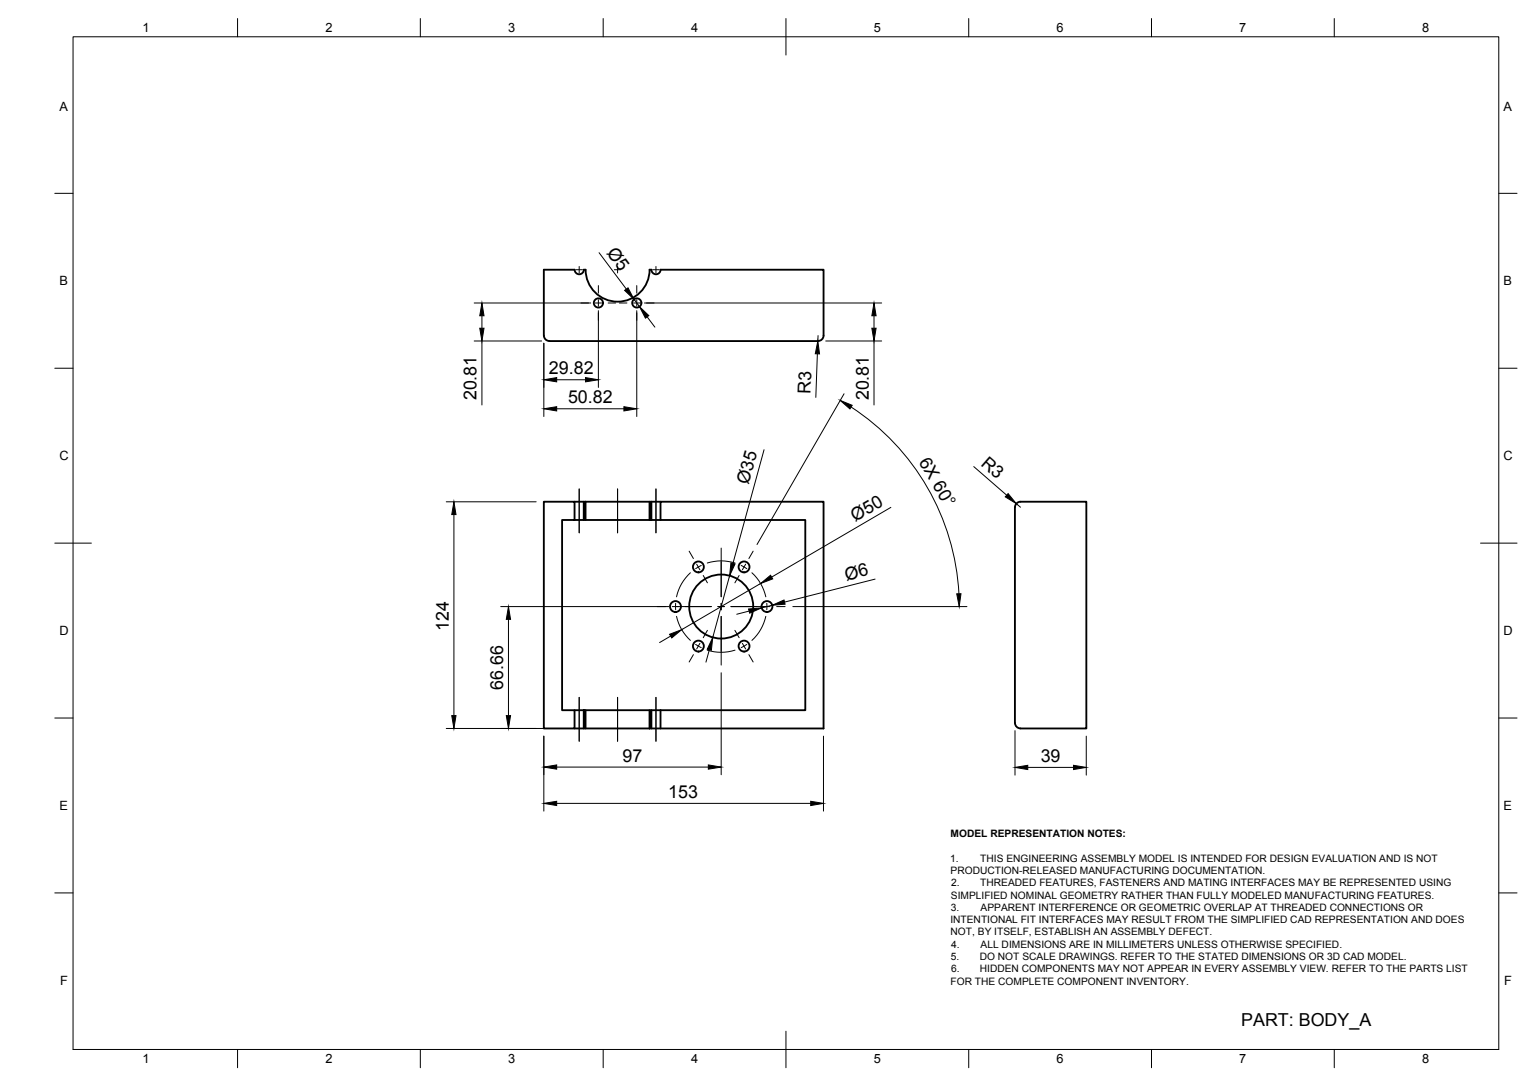
ISO-10303-21;
HEADER;
/* Generated by software containing ST-Developer
 * from STEP Tools, Inc. (www.steptools.com) 
 */

FILE_DESCRIPTION(
/* description */ ('STEP AP214'),
/* implementation_level */ '2;1');

FILE_NAME(
/* name */ 'Body_A.step',
/* time_stamp */ '2026-10-05T13:15:56-07:00',
/* author */ (''),
/* organization */ (''),
/* preprocessor_version */ 'ST-DEVELOPER v20.2',
/* originating_system */ 'Autodesk Translation Framework v15.15.0.0',
/* authorisation */ '');

FILE_SCHEMA (('AUTOMOTIVE_DESIGN { 1 0 10303 214 3 1 1 }'));
ENDSEC;

DATA;
#10=MECHANICAL_DESIGN_GEOMETRIC_PRESENTATION_REPRESENTATION('',(#1345),#37881);
#1321=SHAPE_REPRESENTATION_RELATIONSHIP('SRR','None',#37954,#1333);
#1333=ADVANCED_BREP_SHAPE_REPRESENTATION('',(#1357),#37869);
#1345=STYLED_ITEM('',(#38023),#1357);
#1357=MANIFOLD_SOLID_BREP('Body1',#10819);
#1369=ELLIPSE('',#11034,4.24264068711896,2.99999999999969);
#1370=ELLIPSE('',#11035,4.24264068711823,2.99999999999929);
#1371=ELLIPSE('',#11037,4.24264068711881,2.99999999999963);
#1372=ELLIPSE('',#11039,4.24264068711841,2.99999999999935);
#1377=FACE_BOUND('',#2191,.T.);
#1378=FACE_BOUND('',#2192,.T.);
#1379=FACE_BOUND('',#2195,.T.);
#1380=FACE_BOUND('',#2196,.T.);
#1381=FACE_BOUND('',#2200,.T.);
#1382=FACE_BOUND('',#2201,.T.);
#1383=FACE_BOUND('',#2204,.T.);
#1384=FACE_BOUND('',#2205,.T.);
#1385=FACE_BOUND('',#2208,.T.);
#1386=FACE_BOUND('',#2209,.T.);
#1387=FACE_BOUND('',#2210,.T.);
#1388=FACE_BOUND('',#2211,.T.);
#1389=FACE_BOUND('',#2212,.T.);
#1390=FACE_BOUND('',#2213,.T.);
#1391=FACE_BOUND('',#2214,.T.);
#1392=FACE_BOUND('',#2216,.T.);
#1393=FACE_BOUND('',#2217,.T.);
#1394=FACE_BOUND('',#2218,.T.);
#1395=FACE_BOUND('',#2219,.T.);
#1396=FACE_BOUND('',#2220,.T.);
#1397=FACE_BOUND('',#2221,.T.);
#1398=FACE_BOUND('',#2222,.T.);
#1465=PLANE('',#10999);
#1466=PLANE('',#11000);
#1467=PLANE('',#11001);
#1468=PLANE('',#11002);
#1469=PLANE('',#11003);
#1470=PLANE('',#11004);
#1471=PLANE('',#11008);
#1472=PLANE('',#11009);
#1473=PLANE('',#11013);
#1474=PLANE('',#11014);
#1475=PLANE('',#11015);
#1476=PLANE('',#11019);
#1477=PLANE('',#11020);
#1478=PLANE('',#11024);
#1479=PLANE('',#11025);
#1480=PLANE('',#11026);
#1565=FACE_OUTER_BOUND('',#2174,.T.);
#1566=FACE_OUTER_BOUND('',#2175,.T.);
#1567=FACE_OUTER_BOUND('',#2176,.T.);
#1568=FACE_OUTER_BOUND('',#2177,.T.);
#1569=FACE_OUTER_BOUND('',#2178,.T.);
#1570=FACE_OUTER_BOUND('',#2179,.T.);
#1571=FACE_OUTER_BOUND('',#2180,.T.);
#1572=FACE_OUTER_BOUND('',#2181,.T.);
#1573=FACE_OUTER_BOUND('',#2182,.T.);
#1574=FACE_OUTER_BOUND('',#2183,.T.);
#1575=FACE_OUTER_BOUND('',#2184,.T.);
#1576=FACE_OUTER_BOUND('',#2185,.T.);
#1577=FACE_OUTER_BOUND('',#2186,.T.);
#1578=FACE_OUTER_BOUND('',#2187,.T.);
#1579=FACE_OUTER_BOUND('',#2188,.T.);
#1580=FACE_OUTER_BOUND('',#2189,.T.);
#1581=FACE_OUTER_BOUND('',#2190,.T.);
#1582=FACE_OUTER_BOUND('',#2193,.T.);
#1583=FACE_OUTER_BOUND('',#2194,.T.);
#1584=FACE_OUTER_BOUND('',#2197,.T.);
#1585=FACE_OUTER_BOUND('',#2198,.T.);
#1586=FACE_OUTER_BOUND('',#2199,.T.);
#1587=FACE_OUTER_BOUND('',#2202,.T.);
#1588=FACE_OUTER_BOUND('',#2203,.T.);
#1589=FACE_OUTER_BOUND('',#2206,.T.);
#1590=FACE_OUTER_BOUND('',#2207,.T.);
#1591=FACE_OUTER_BOUND('',#2215,.T.);
#1592=FACE_OUTER_BOUND('',#2223,.T.);
#1593=FACE_OUTER_BOUND('',#2224,.T.);
#1594=FACE_OUTER_BOUND('',#2225,.T.);
#1595=FACE_OUTER_BOUND('',#2226,.T.);
#1596=FACE_OUTER_BOUND('',#2227,.T.);
#1597=FACE_OUTER_BOUND('',#2228,.T.);
#1598=FACE_OUTER_BOUND('',#2229,.T.);
#1599=FACE_OUTER_BOUND('',#2230,.T.);
#1600=FACE_OUTER_BOUND('',#2231,.T.);
#1601=FACE_OUTER_BOUND('',#2232,.T.);
#2174=EDGE_LOOP('',(#6725,#6726,#6727,#6728));
#2175=EDGE_LOOP('',(#6729,#6730,#6731,#6732));
#2176=EDGE_LOOP('',(#6733,#6734,#6735,#6736));
#2177=EDGE_LOOP('',(#6737,#6738,#6739,#6740));
#2178=EDGE_LOOP('',(#6741,#6742,#6743,#6744));
#2179=EDGE_LOOP('',(#6745,#6746,#6747,#6748));
#2180=EDGE_LOOP('',(#6749,#6750,#6751,#6752));
#2181=EDGE_LOOP('',(#6753,#6754,#6755,#6756));
#2182=EDGE_LOOP('',(#6757,#6758,#6759,#6760));
#2183=EDGE_LOOP('',(#6761,#6762,#6763,#6764));
#2184=EDGE_LOOP('',(#6765,#6766,#6767,#6768));
#2185=EDGE_LOOP('',(#6769,#6770,#6771,#6772,#6773,#6774,#6775,#6776));
#2186=EDGE_LOOP('',(#6777,#6778,#6779,#6780));
#2187=EDGE_LOOP('',(#6781,#6782,#6783,#6784));
#2188=EDGE_LOOP('',(#6785,#6786,#6787,#6788));
#2189=EDGE_LOOP('',(#6789,#6790,#6791,#6792));
#2190=EDGE_LOOP('',(#6793,#6794,#6795,#6796,#6797,#6798,#6799,#6800,#6801,
#6802));
#2191=EDGE_LOOP('',(#6803));
#2192=EDGE_LOOP('',(#6804));
#2193=EDGE_LOOP('',(#6805,#6806,#6807,#6808,#6809,#6810,#6811,#6812));
#2194=EDGE_LOOP('',(#6813,#6814,#6815,#6816,#6817,#6818,#6819,#6820,#6821,
#6822));
#2195=EDGE_LOOP('',(#6823));
#2196=EDGE_LOOP('',(#6824));
#2197=EDGE_LOOP('',(#6825,#6826,#6827,#6828));
#2198=EDGE_LOOP('',(#6829,#6830,#6831,#6832));
#2199=EDGE_LOOP('',(#6833,#6834,#6835,#6836,#6837,#6838,#6839,#6840,#6841,
#6842));
#2200=EDGE_LOOP('',(#6843));
#2201=EDGE_LOOP('',(#6844));
#2202=EDGE_LOOP('',(#6845,#6846,#6847,#6848));
#2203=EDGE_LOOP('',(#6849,#6850,#6851,#6852,#6853,#6854,#6855,#6856,#6857,
#6858));
#2204=EDGE_LOOP('',(#6859));
#2205=EDGE_LOOP('',(#6860));
#2206=EDGE_LOOP('',(#6861,#6862,#6863,#6864));
#2207=EDGE_LOOP('',(#6865,#6866,#6867,#6868));
#2208=EDGE_LOOP('',(#6869));
#2209=EDGE_LOOP('',(#6870));
#2210=EDGE_LOOP('',(#6871));
#2211=EDGE_LOOP('',(#6872));
#2212=EDGE_LOOP('',(#6873));
#2213=EDGE_LOOP('',(#6874));
#2214=EDGE_LOOP('',(#6875));
#2215=EDGE_LOOP('',(#6876,#6877,#6878,#6879));
#2216=EDGE_LOOP('',(#6880));
#2217=EDGE_LOOP('',(#6881));
#2218=EDGE_LOOP('',(#6882));
#2219=EDGE_LOOP('',(#6883));
#2220=EDGE_LOOP('',(#6884));
#2221=EDGE_LOOP('',(#6885));
#2222=EDGE_LOOP('',(#6886));
#2223=EDGE_LOOP('',(#6887,#6888,#6889,#6890));
#2224=EDGE_LOOP('',(#6891,#6892,#6893,#6894));
#2225=EDGE_LOOP('',(#6895,#6896,#6897,#6898));
#2226=EDGE_LOOP('',(#6899,#6900,#6901,#6902));
#2227=EDGE_LOOP('',(#6903,#6904,#6905,#6906));
#2228=EDGE_LOOP('',(#6907,#6908,#6909,#6910));
#2229=EDGE_LOOP('',(#6911,#6912,#6913,#6914));
#2230=EDGE_LOOP('',(#6915,#6916,#6917,#6918));
#2231=EDGE_LOOP('',(#6919,#6920,#6921,#6922));
#2232=EDGE_LOOP('',(#6923,#6924,#6925,#6926));
#2871=LINE('',#14049,#3172);
#2872=LINE('',#14055,#3173);
#2873=LINE('',#14061,#3174);
#2874=LINE('',#14067,#3175);
#2875=LINE('',#14073,#3176);
#2876=LINE('',#14079,#3177);
#2877=LINE('',#14085,#3178);
#2878=LINE('',#14091,#3179);
#2879=LINE('',#14097,#3180);
#2880=LINE('',#14103,#3181);
#2881=LINE('',#14109,#3182);
#2882=LINE('',#14114,#3183);
#2883=LINE('',#14116,#3184);
#2884=LINE('',#14118,#3185);
#2885=LINE('',#14120,#3186);
#2886=LINE('',#14122,#3187);
#2887=LINE('',#14124,#3188);
#2888=LINE('',#14126,#3189);
#2889=LINE('',#14127,#3190);
#2890=LINE('',#14131,#3191);
#2891=LINE('',#14133,#3192);
#2892=LINE('',#14135,#3193);
#2893=LINE('',#14136,#3194);
#2894=LINE('',#14140,#3195);
#2895=LINE('',#14142,#3196);
#2896=LINE('',#14144,#3197);
#2897=LINE('',#14145,#3198);
#2898=LINE('',#14149,#3199);
#2899=LINE('',#14151,#3200);
#2900=LINE('',#14153,#3201);
#2901=LINE('',#14154,#3202);
#2902=LINE('',#14158,#3203);
#2903=LINE('',#14160,#3204);
#2904=LINE('',#14162,#3205);
#2905=LINE('',#14163,#3206);
#2906=LINE('',#14166,#3207);
#2907=LINE('',#14168,#3208);
#2908=LINE('',#14170,#3209);
#2909=LINE('',#14172,#3210);
#2910=LINE('',#14178,#3211);
#2911=LINE('',#14180,#3212);
#2912=LINE('',#14182,#3213);
#2913=LINE('',#14184,#3214);
#2914=LINE('',#14186,#3215);
#2915=LINE('',#14188,#3216);
#2916=LINE('',#14189,#3217);
#2917=LINE('',#14192,#3218);
#2918=LINE('',#14194,#3219);
#2919=LINE('',#14195,#3220);
#2920=LINE('',#14200,#3221);
#2921=LINE('',#14202,#3222);
#2922=LINE('',#14208,#3223);
#2923=LINE('',#14210,#3224);
#2924=LINE('',#14211,#3225);
#2925=LINE('',#14214,#3226);
#2926=LINE('',#14215,#3227);
#2927=LINE('',#14219,#3228);
#2928=LINE('',#14220,#3229);
#2929=LINE('',#14224,#3230);
#2930=LINE('',#14229,#3231);
#2931=LINE('',#14231,#3232);
#2932=LINE('',#14233,#3233);
#2933=LINE('',#14234,#3234);
#3172=VECTOR('',#11898,2.5);
#3173=VECTOR('',#11905,2.5);
#3174=VECTOR('',#11912,2.5);
#3175=VECTOR('',#11919,2.5);
#3176=VECTOR('',#11926,3.);
#3177=VECTOR('',#11933,2.99999999999999);
#3178=VECTOR('',#11940,3.);
#3179=VECTOR('',#11947,3.);
#3180=VECTOR('',#11954,3.);
#3181=VECTOR('',#11961,3.);
#3182=VECTOR('',#11968,17.5);
#3183=VECTOR('',#11973,1000.);
#3184=VECTOR('',#11974,1000.);
#3185=VECTOR('',#11975,1000.);
#3186=VECTOR('',#11976,1000.);
#3187=VECTOR('',#11977,1000.);
#3188=VECTOR('',#11978,1000.);
#3189=VECTOR('',#11979,1000.);
#3190=VECTOR('',#11980,1000.);
#3191=VECTOR('',#11983,1000.);
#3192=VECTOR('',#11984,1000.);
#3193=VECTOR('',#11985,1000.);
#3194=VECTOR('',#11986,1000.);
#3195=VECTOR('',#11989,1000.);
#3196=VECTOR('',#11990,1000.);
#3197=VECTOR('',#11991,1000.);
#3198=VECTOR('',#11992,1000.);
#3199=VECTOR('',#11995,1000.);
#3200=VECTOR('',#11996,1000.);
#3201=VECTOR('',#11997,1000.);
#3202=VECTOR('',#11998,1000.);
#3203=VECTOR('',#12001,1000.);
#3204=VECTOR('',#12002,1000.);
#3205=VECTOR('',#12003,1000.);
#3206=VECTOR('',#12004,1000.);
#3207=VECTOR('',#12007,1000.);
#3208=VECTOR('',#12008,1000.);
#3209=VECTOR('',#12009,1000.);
#3210=VECTOR('',#12010,1000.);
#3211=VECTOR('',#12019,1000.);
#3212=VECTOR('',#12020,1000.);
#3213=VECTOR('',#12021,1000.);
#3214=VECTOR('',#12022,1000.);
#3215=VECTOR('',#12023,1000.);
#3216=VECTOR('',#12024,1000.);
#3217=VECTOR('',#12025,1000.);
#3218=VECTOR('',#12028,1000.);
#3219=VECTOR('',#12029,1000.);
#3220=VECTOR('',#12030,1000.);
#3221=VECTOR('',#12039,1000.);
#3222=VECTOR('',#12042,1000.);
#3223=VECTOR('',#12051,1000.);
#3224=VECTOR('',#12052,1000.);
#3225=VECTOR('',#12053,1000.);
#3226=VECTOR('',#12056,1000.);
#3227=VECTOR('',#12057,1000.);
#3228=VECTOR('',#12062,1000.);
#3229=VECTOR('',#12063,1000.);
#3230=VECTOR('',#12070,1000.);
#3231=VECTOR('',#12075,1000.);
#3232=VECTOR('',#12076,1000.);
#3233=VECTOR('',#12077,1000.);
#3234=VECTOR('',#12078,1000.);
#3473=CIRCLE('',#10967,2.5);
#3474=CIRCLE('',#10968,2.5);
#3475=CIRCLE('',#10970,2.5);
#3476=CIRCLE('',#10971,2.5);
#3477=CIRCLE('',#10973,2.5);
#3478=CIRCLE('',#10974,2.5);
#3479=CIRCLE('',#10976,2.5);
#3480=CIRCLE('',#10977,2.5);
#3481=CIRCLE('',#10979,3.);
#3482=CIRCLE('',#10980,3.);
#3483=CIRCLE('',#10982,2.99999999999999);
#3484=CIRCLE('',#10983,2.99999999999999);
#3485=CIRCLE('',#10985,3.);
#3486=CIRCLE('',#10986,3.);
#3487=CIRCLE('',#10988,3.);
#3488=CIRCLE('',#10989,3.);
#3489=CIRCLE('',#10991,3.);
#3490=CIRCLE('',#10992,3.);
#3491=CIRCLE('',#10994,3.);
#3492=CIRCLE('',#10995,3.);
#3493=CIRCLE('',#10997,17.5);
#3494=CIRCLE('',#10998,17.5);
#3495=CIRCLE('',#11005,2.50000000000001);
#3496=CIRCLE('',#11006,17.5);
#3497=CIRCLE('',#11007,2.5);
#3498=CIRCLE('',#11010,2.5);
#3499=CIRCLE('',#11011,17.5);
#3500=CIRCLE('',#11012,2.50000000000001);
#3501=CIRCLE('',#11016,2.5);
#3502=CIRCLE('',#11017,17.5);
#3503=CIRCLE('',#11018,2.50000000000001);
#3504=CIRCLE('',#11021,2.5);
#3505=CIRCLE('',#11022,2.50000000000001);
#3506=CIRCLE('',#11023,17.5);
#3998=VERTEX_POINT('',#14046);
#3999=VERTEX_POINT('',#14048);
#4000=VERTEX_POINT('',#14052);
#4001=VERTEX_POINT('',#14054);
#4002=VERTEX_POINT('',#14058);
#4003=VERTEX_POINT('',#14060);
#4004=VERTEX_POINT('',#14064);
#4005=VERTEX_POINT('',#14066);
#4006=VERTEX_POINT('',#14070);
#4007=VERTEX_POINT('',#14072);
#4008=VERTEX_POINT('',#14076);
#4009=VERTEX_POINT('',#14078);
#4010=VERTEX_POINT('',#14082);
#4011=VERTEX_POINT('',#14084);
#4012=VERTEX_POINT('',#14088);
#4013=VERTEX_POINT('',#14090);
#4014=VERTEX_POINT('',#14094);
#4015=VERTEX_POINT('',#14096);
#4016=VERTEX_POINT('',#14100);
#4017=VERTEX_POINT('',#14102);
#4018=VERTEX_POINT('',#14106);
#4019=VERTEX_POINT('',#14108);
#4020=VERTEX_POINT('',#14112);
#4021=VERTEX_POINT('',#14113);
#4022=VERTEX_POINT('',#14115);
#4023=VERTEX_POINT('',#14117);
#4024=VERTEX_POINT('',#14119);
#4025=VERTEX_POINT('',#14121);
#4026=VERTEX_POINT('',#14123);
#4027=VERTEX_POINT('',#14125);
#4028=VERTEX_POINT('',#14129);
#4029=VERTEX_POINT('',#14130);
#4030=VERTEX_POINT('',#14132);
#4031=VERTEX_POINT('',#14134);
#4032=VERTEX_POINT('',#14138);
#4033=VERTEX_POINT('',#14139);
#4034=VERTEX_POINT('',#14141);
#4035=VERTEX_POINT('',#14143);
#4036=VERTEX_POINT('',#14147);
#4037=VERTEX_POINT('',#14148);
#4038=VERTEX_POINT('',#14150);
#4039=VERTEX_POINT('',#14152);
#4040=VERTEX_POINT('',#14156);
#4041=VERTEX_POINT('',#14157);
#4042=VERTEX_POINT('',#14159);
#4043=VERTEX_POINT('',#14161);
#4044=VERTEX_POINT('',#14165);
#4045=VERTEX_POINT('',#14167);
#4046=VERTEX_POINT('',#14169);
#4047=VERTEX_POINT('',#14171);
#4048=VERTEX_POINT('',#14177);
#4049=VERTEX_POINT('',#14179);
#4050=VERTEX_POINT('',#14181);
#4051=VERTEX_POINT('',#14183);
#4052=VERTEX_POINT('',#14185);
#4053=VERTEX_POINT('',#14187);
#4054=VERTEX_POINT('',#14191);
#4055=VERTEX_POINT('',#14193);
#4056=VERTEX_POINT('',#14207);
#4057=VERTEX_POINT('',#14209);
#4058=VERTEX_POINT('',#14213);
#4059=VERTEX_POINT('',#14218);
#4060=VERTEX_POINT('',#14227);
#4061=VERTEX_POINT('',#14228);
#4062=VERTEX_POINT('',#14230);
#4063=VERTEX_POINT('',#14232);
#5073=EDGE_CURVE('',#3998,#3998,#3473,.T.);
#5074=EDGE_CURVE('',#3998,#3999,#2871,.T.);
#5075=EDGE_CURVE('',#3999,#3999,#3474,.T.);
#5076=EDGE_CURVE('',#4000,#4000,#3475,.T.);
#5077=EDGE_CURVE('',#4000,#4001,#2872,.T.);
#5078=EDGE_CURVE('',#4001,#4001,#3476,.T.);
#5079=EDGE_CURVE('',#4002,#4002,#3477,.T.);
#5080=EDGE_CURVE('',#4002,#4003,#2873,.T.);
#5081=EDGE_CURVE('',#4003,#4003,#3478,.T.);
#5082=EDGE_CURVE('',#4004,#4004,#3479,.T.);
#5083=EDGE_CURVE('',#4004,#4005,#2874,.T.);
#5084=EDGE_CURVE('',#4005,#4005,#3480,.T.);
#5085=EDGE_CURVE('',#4006,#4006,#3481,.T.);
#5086=EDGE_CURVE('',#4006,#4007,#2875,.T.);
#5087=EDGE_CURVE('',#4007,#4007,#3482,.T.);
#5088=EDGE_CURVE('',#4008,#4008,#3483,.T.);
#5089=EDGE_CURVE('',#4008,#4009,#2876,.T.);
#5090=EDGE_CURVE('',#4009,#4009,#3484,.T.);
#5091=EDGE_CURVE('',#4010,#4010,#3485,.T.);
#5092=EDGE_CURVE('',#4010,#4011,#2877,.T.);
#5093=EDGE_CURVE('',#4011,#4011,#3486,.T.);
#5094=EDGE_CURVE('',#4012,#4012,#3487,.T.);
#5095=EDGE_CURVE('',#4012,#4013,#2878,.T.);
#5096=EDGE_CURVE('',#4013,#4013,#3488,.T.);
#5097=EDGE_CURVE('',#4014,#4014,#3489,.T.);
#5098=EDGE_CURVE('',#4014,#4015,#2879,.T.);
#5099=EDGE_CURVE('',#4015,#4015,#3490,.T.);
#5100=EDGE_CURVE('',#4016,#4016,#3491,.T.);
#5101=EDGE_CURVE('',#4016,#4017,#2880,.T.);
#5102=EDGE_CURVE('',#4017,#4017,#3492,.T.);
#5103=EDGE_CURVE('',#4018,#4018,#3493,.T.);
#5104=EDGE_CURVE('',#4018,#4019,#2881,.T.);
#5105=EDGE_CURVE('',#4019,#4019,#3494,.T.);
#5106=EDGE_CURVE('',#4020,#4021,#2882,.T.);
#5107=EDGE_CURVE('',#4022,#4020,#2883,.T.);
#5108=EDGE_CURVE('',#4023,#4022,#2884,.T.);
#5109=EDGE_CURVE('',#4024,#4023,#2885,.T.);
#5110=EDGE_CURVE('',#4025,#4024,#2886,.T.);
#5111=EDGE_CURVE('',#4025,#4026,#2887,.T.);
#5112=EDGE_CURVE('',#4026,#4027,#2888,.T.);
#5113=EDGE_CURVE('',#4027,#4021,#2889,.T.);
#5114=EDGE_CURVE('',#4028,#4029,#2890,.T.);
#5115=EDGE_CURVE('',#4030,#4028,#2891,.T.);
#5116=EDGE_CURVE('',#4031,#4030,#2892,.T.);
#5117=EDGE_CURVE('',#4031,#4029,#2893,.T.);
#5118=EDGE_CURVE('',#4032,#4033,#2894,.T.);
#5119=EDGE_CURVE('',#4032,#4034,#2895,.T.);
#5120=EDGE_CURVE('',#4035,#4034,#2896,.T.);
#5121=EDGE_CURVE('',#4033,#4035,#2897,.T.);
#5122=EDGE_CURVE('',#4036,#4037,#2898,.T.);
#5123=EDGE_CURVE('',#4038,#4036,#2899,.T.);
#5124=EDGE_CURVE('',#4039,#4038,#2900,.T.);
#5125=EDGE_CURVE('',#4039,#4037,#2901,.T.);
#5126=EDGE_CURVE('',#4040,#4041,#2902,.T.);
#5127=EDGE_CURVE('',#4040,#4042,#2903,.T.);
#5128=EDGE_CURVE('',#4043,#4042,#2904,.T.);
#5129=EDGE_CURVE('',#4041,#4043,#2905,.T.);
#5130=EDGE_CURVE('',#4044,#4023,#2906,.T.);
#5131=EDGE_CURVE('',#4044,#4045,#2907,.T.);
#5132=EDGE_CURVE('',#4045,#4046,#2908,.T.);
#5133=EDGE_CURVE('',#4046,#4047,#2909,.T.);
#5134=EDGE_CURVE('',#4033,#4047,#3495,.T.);
#5135=EDGE_CURVE('',#4030,#4035,#3496,.T.);
#5136=EDGE_CURVE('',#4024,#4028,#3497,.T.);
#5137=EDGE_CURVE('',#4047,#4048,#2910,.T.);
#5138=EDGE_CURVE('',#4049,#4046,#2911,.T.);
#5139=EDGE_CURVE('',#4050,#4049,#2912,.T.);
#5140=EDGE_CURVE('',#4051,#4050,#2913,.T.);
#5141=EDGE_CURVE('',#4051,#4052,#2914,.T.);
#5142=EDGE_CURVE('',#4052,#4053,#2915,.T.);
#5143=EDGE_CURVE('',#4053,#4048,#2916,.T.);
#5144=EDGE_CURVE('',#4054,#4049,#2917,.T.);
#5145=EDGE_CURVE('',#4054,#4055,#2918,.T.);
#5146=EDGE_CURVE('',#4055,#4022,#2919,.T.);
#5147=EDGE_CURVE('',#4020,#4041,#3498,.T.);
#5148=EDGE_CURVE('',#4043,#4038,#3499,.T.);
#5149=EDGE_CURVE('',#4036,#4050,#3500,.T.);
#5150=EDGE_CURVE('',#4045,#4054,#2920,.T.);
#5151=EDGE_CURVE('',#4055,#4044,#2921,.T.);
#5152=EDGE_CURVE('',#4029,#4025,#3501,.T.);
#5153=EDGE_CURVE('',#4034,#4031,#3502,.T.);
#5154=EDGE_CURVE('',#4048,#4032,#3503,.T.);
#5155=EDGE_CURVE('',#4056,#4053,#2922,.T.);
#5156=EDGE_CURVE('',#4056,#4057,#2923,.T.);
#5157=EDGE_CURVE('',#4057,#4026,#2924,.T.);
#5158=EDGE_CURVE('',#4057,#4058,#2925,.T.);
#5159=EDGE_CURVE('',#4058,#4027,#2926,.T.);
#5160=EDGE_CURVE('',#4021,#4040,#3504,.T.);
#5161=EDGE_CURVE('',#4058,#4059,#2927,.T.);
#5162=EDGE_CURVE('',#4059,#4052,#2928,.T.);
#5163=EDGE_CURVE('',#4037,#4051,#3505,.T.);
#5164=EDGE_CURVE('',#4042,#4039,#3506,.T.);
#5165=EDGE_CURVE('',#4059,#4056,#2929,.T.);
#5166=EDGE_CURVE('',#4060,#4061,#2930,.T.);
#5167=EDGE_CURVE('',#4061,#4062,#2931,.T.);
#5168=EDGE_CURVE('',#4062,#4063,#2932,.T.);
#5169=EDGE_CURVE('',#4063,#4060,#2933,.T.);
#5170=EDGE_CURVE('',#4045,#4063,#1369,.T.);
#5171=EDGE_CURVE('',#4060,#4044,#1370,.T.);
#5172=EDGE_CURVE('',#4061,#4055,#1371,.T.);
#5173=EDGE_CURVE('',#4054,#4062,#1372,.T.);
#6725=ORIENTED_EDGE('',*,*,#5073,.T.);
#6726=ORIENTED_EDGE('',*,*,#5074,.T.);
#6727=ORIENTED_EDGE('',*,*,#5075,.T.);
#6728=ORIENTED_EDGE('',*,*,#5074,.F.);
#6729=ORIENTED_EDGE('',*,*,#5076,.T.);
#6730=ORIENTED_EDGE('',*,*,#5077,.T.);
#6731=ORIENTED_EDGE('',*,*,#5078,.T.);
#6732=ORIENTED_EDGE('',*,*,#5077,.F.);
#6733=ORIENTED_EDGE('',*,*,#5079,.F.);
#6734=ORIENTED_EDGE('',*,*,#5080,.T.);
#6735=ORIENTED_EDGE('',*,*,#5081,.T.);
#6736=ORIENTED_EDGE('',*,*,#5080,.F.);
#6737=ORIENTED_EDGE('',*,*,#5082,.F.);
#6738=ORIENTED_EDGE('',*,*,#5083,.T.);
#6739=ORIENTED_EDGE('',*,*,#5084,.T.);
#6740=ORIENTED_EDGE('',*,*,#5083,.F.);
#6741=ORIENTED_EDGE('',*,*,#5085,.F.);
#6742=ORIENTED_EDGE('',*,*,#5086,.T.);
#6743=ORIENTED_EDGE('',*,*,#5087,.T.);
#6744=ORIENTED_EDGE('',*,*,#5086,.F.);
#6745=ORIENTED_EDGE('',*,*,#5088,.F.);
#6746=ORIENTED_EDGE('',*,*,#5089,.T.);
#6747=ORIENTED_EDGE('',*,*,#5090,.T.);
#6748=ORIENTED_EDGE('',*,*,#5089,.F.);
#6749=ORIENTED_EDGE('',*,*,#5091,.F.);
#6750=ORIENTED_EDGE('',*,*,#5092,.T.);
#6751=ORIENTED_EDGE('',*,*,#5093,.T.);
#6752=ORIENTED_EDGE('',*,*,#5092,.F.);
#6753=ORIENTED_EDGE('',*,*,#5094,.F.);
#6754=ORIENTED_EDGE('',*,*,#5095,.T.);
#6755=ORIENTED_EDGE('',*,*,#5096,.T.);
#6756=ORIENTED_EDGE('',*,*,#5095,.F.);
#6757=ORIENTED_EDGE('',*,*,#5097,.F.);
#6758=ORIENTED_EDGE('',*,*,#5098,.T.);
#6759=ORIENTED_EDGE('',*,*,#5099,.T.);
#6760=ORIENTED_EDGE('',*,*,#5098,.F.);
#6761=ORIENTED_EDGE('',*,*,#5100,.F.);
#6762=ORIENTED_EDGE('',*,*,#5101,.T.);
#6763=ORIENTED_EDGE('',*,*,#5102,.T.);
#6764=ORIENTED_EDGE('',*,*,#5101,.F.);
#6765=ORIENTED_EDGE('',*,*,#5103,.F.);
#6766=ORIENTED_EDGE('',*,*,#5104,.T.);
#6767=ORIENTED_EDGE('',*,*,#5105,.T.);
#6768=ORIENTED_EDGE('',*,*,#5104,.F.);
#6769=ORIENTED_EDGE('',*,*,#5106,.F.);
#6770=ORIENTED_EDGE('',*,*,#5107,.F.);
#6771=ORIENTED_EDGE('',*,*,#5108,.F.);
#6772=ORIENTED_EDGE('',*,*,#5109,.F.);
#6773=ORIENTED_EDGE('',*,*,#5110,.F.);
#6774=ORIENTED_EDGE('',*,*,#5111,.T.);
#6775=ORIENTED_EDGE('',*,*,#5112,.T.);
#6776=ORIENTED_EDGE('',*,*,#5113,.T.);
#6777=ORIENTED_EDGE('',*,*,#5114,.F.);
#6778=ORIENTED_EDGE('',*,*,#5115,.F.);
#6779=ORIENTED_EDGE('',*,*,#5116,.F.);
#6780=ORIENTED_EDGE('',*,*,#5117,.T.);
#6781=ORIENTED_EDGE('',*,*,#5118,.F.);
#6782=ORIENTED_EDGE('',*,*,#5119,.T.);
#6783=ORIENTED_EDGE('',*,*,#5120,.F.);
#6784=ORIENTED_EDGE('',*,*,#5121,.F.);
#6785=ORIENTED_EDGE('',*,*,#5122,.F.);
#6786=ORIENTED_EDGE('',*,*,#5123,.F.);
#6787=ORIENTED_EDGE('',*,*,#5124,.F.);
#6788=ORIENTED_EDGE('',*,*,#5125,.T.);
#6789=ORIENTED_EDGE('',*,*,#5126,.F.);
#6790=ORIENTED_EDGE('',*,*,#5127,.T.);
#6791=ORIENTED_EDGE('',*,*,#5128,.F.);
#6792=ORIENTED_EDGE('',*,*,#5129,.F.);
#6793=ORIENTED_EDGE('',*,*,#5130,.F.);
#6794=ORIENTED_EDGE('',*,*,#5131,.T.);
#6795=ORIENTED_EDGE('',*,*,#5132,.T.);
#6796=ORIENTED_EDGE('',*,*,#5133,.T.);
#6797=ORIENTED_EDGE('',*,*,#5134,.F.);
#6798=ORIENTED_EDGE('',*,*,#5121,.T.);
#6799=ORIENTED_EDGE('',*,*,#5135,.F.);
#6800=ORIENTED_EDGE('',*,*,#5115,.T.);
#6801=ORIENTED_EDGE('',*,*,#5136,.F.);
#6802=ORIENTED_EDGE('',*,*,#5109,.T.);
#6803=ORIENTED_EDGE('',*,*,#5078,.F.);
#6804=ORIENTED_EDGE('',*,*,#5075,.F.);
#6805=ORIENTED_EDGE('',*,*,#5137,.F.);
#6806=ORIENTED_EDGE('',*,*,#5133,.F.);
#6807=ORIENTED_EDGE('',*,*,#5138,.F.);
#6808=ORIENTED_EDGE('',*,*,#5139,.F.);
#6809=ORIENTED_EDGE('',*,*,#5140,.F.);
#6810=ORIENTED_EDGE('',*,*,#5141,.T.);
#6811=ORIENTED_EDGE('',*,*,#5142,.T.);
#6812=ORIENTED_EDGE('',*,*,#5143,.T.);
#6813=ORIENTED_EDGE('',*,*,#5144,.F.);
#6814=ORIENTED_EDGE('',*,*,#5145,.T.);
#6815=ORIENTED_EDGE('',*,*,#5146,.T.);
#6816=ORIENTED_EDGE('',*,*,#5107,.T.);
#6817=ORIENTED_EDGE('',*,*,#5147,.T.);
#6818=ORIENTED_EDGE('',*,*,#5129,.T.);
#6819=ORIENTED_EDGE('',*,*,#5148,.T.);
#6820=ORIENTED_EDGE('',*,*,#5123,.T.);
#6821=ORIENTED_EDGE('',*,*,#5149,.T.);
#6822=ORIENTED_EDGE('',*,*,#5139,.T.);
#6823=ORIENTED_EDGE('',*,*,#5079,.T.);
#6824=ORIENTED_EDGE('',*,*,#5082,.T.);
#6825=ORIENTED_EDGE('',*,*,#5132,.F.);
#6826=ORIENTED_EDGE('',*,*,#5150,.T.);
#6827=ORIENTED_EDGE('',*,*,#5144,.T.);
#6828=ORIENTED_EDGE('',*,*,#5138,.T.);
#6829=ORIENTED_EDGE('',*,*,#5146,.F.);
#6830=ORIENTED_EDGE('',*,*,#5151,.T.);
#6831=ORIENTED_EDGE('',*,*,#5130,.T.);
#6832=ORIENTED_EDGE('',*,*,#5108,.T.);
#6833=ORIENTED_EDGE('',*,*,#5152,.F.);
#6834=ORIENTED_EDGE('',*,*,#5117,.F.);
#6835=ORIENTED_EDGE('',*,*,#5153,.F.);
#6836=ORIENTED_EDGE('',*,*,#5119,.F.);
#6837=ORIENTED_EDGE('',*,*,#5154,.F.);
#6838=ORIENTED_EDGE('',*,*,#5143,.F.);
#6839=ORIENTED_EDGE('',*,*,#5155,.F.);
#6840=ORIENTED_EDGE('',*,*,#5156,.T.);
#6841=ORIENTED_EDGE('',*,*,#5157,.T.);
#6842=ORIENTED_EDGE('',*,*,#5111,.F.);
#6843=ORIENTED_EDGE('',*,*,#5073,.F.);
#6844=ORIENTED_EDGE('',*,*,#5076,.F.);
#6845=ORIENTED_EDGE('',*,*,#5112,.F.);
#6846=ORIENTED_EDGE('',*,*,#5157,.F.);
#6847=ORIENTED_EDGE('',*,*,#5158,.T.);
#6848=ORIENTED_EDGE('',*,*,#5159,.T.);
#6849=ORIENTED_EDGE('',*,*,#5160,.F.);
#6850=ORIENTED_EDGE('',*,*,#5113,.F.);
#6851=ORIENTED_EDGE('',*,*,#5159,.F.);
#6852=ORIENTED_EDGE('',*,*,#5161,.T.);
#6853=ORIENTED_EDGE('',*,*,#5162,.T.);
#6854=ORIENTED_EDGE('',*,*,#5141,.F.);
#6855=ORIENTED_EDGE('',*,*,#5163,.F.);
#6856=ORIENTED_EDGE('',*,*,#5125,.F.);
#6857=ORIENTED_EDGE('',*,*,#5164,.F.);
#6858=ORIENTED_EDGE('',*,*,#5127,.F.);
#6859=ORIENTED_EDGE('',*,*,#5081,.F.);
#6860=ORIENTED_EDGE('',*,*,#5084,.F.);
#6861=ORIENTED_EDGE('',*,*,#5142,.F.);
#6862=ORIENTED_EDGE('',*,*,#5162,.F.);
#6863=ORIENTED_EDGE('',*,*,#5165,.T.);
#6864=ORIENTED_EDGE('',*,*,#5155,.T.);
#6865=ORIENTED_EDGE('',*,*,#5156,.F.);
#6866=ORIENTED_EDGE('',*,*,#5165,.F.);
#6867=ORIENTED_EDGE('',*,*,#5161,.F.);
#6868=ORIENTED_EDGE('',*,*,#5158,.F.);
#6869=ORIENTED_EDGE('',*,*,#5085,.T.);
#6870=ORIENTED_EDGE('',*,*,#5088,.T.);
#6871=ORIENTED_EDGE('',*,*,#5091,.T.);
#6872=ORIENTED_EDGE('',*,*,#5094,.T.);
#6873=ORIENTED_EDGE('',*,*,#5097,.T.);
#6874=ORIENTED_EDGE('',*,*,#5100,.T.);
#6875=ORIENTED_EDGE('',*,*,#5103,.T.);
#6876=ORIENTED_EDGE('',*,*,#5166,.T.);
#6877=ORIENTED_EDGE('',*,*,#5167,.T.);
#6878=ORIENTED_EDGE('',*,*,#5168,.T.);
#6879=ORIENTED_EDGE('',*,*,#5169,.T.);
#6880=ORIENTED_EDGE('',*,*,#5087,.F.);
#6881=ORIENTED_EDGE('',*,*,#5090,.F.);
#6882=ORIENTED_EDGE('',*,*,#5093,.F.);
#6883=ORIENTED_EDGE('',*,*,#5096,.F.);
#6884=ORIENTED_EDGE('',*,*,#5099,.F.);
#6885=ORIENTED_EDGE('',*,*,#5102,.F.);
#6886=ORIENTED_EDGE('',*,*,#5105,.F.);
#6887=ORIENTED_EDGE('',*,*,#5128,.T.);
#6888=ORIENTED_EDGE('',*,*,#5164,.T.);
#6889=ORIENTED_EDGE('',*,*,#5124,.T.);
#6890=ORIENTED_EDGE('',*,*,#5148,.F.);
#6891=ORIENTED_EDGE('',*,*,#5122,.T.);
#6892=ORIENTED_EDGE('',*,*,#5163,.T.);
#6893=ORIENTED_EDGE('',*,*,#5140,.T.);
#6894=ORIENTED_EDGE('',*,*,#5149,.F.);
#6895=ORIENTED_EDGE('',*,*,#5106,.T.);
#6896=ORIENTED_EDGE('',*,*,#5160,.T.);
#6897=ORIENTED_EDGE('',*,*,#5126,.T.);
#6898=ORIENTED_EDGE('',*,*,#5147,.F.);
#6899=ORIENTED_EDGE('',*,*,#5116,.T.);
#6900=ORIENTED_EDGE('',*,*,#5135,.T.);
#6901=ORIENTED_EDGE('',*,*,#5120,.T.);
#6902=ORIENTED_EDGE('',*,*,#5153,.T.);
#6903=ORIENTED_EDGE('',*,*,#5118,.T.);
#6904=ORIENTED_EDGE('',*,*,#5134,.T.);
#6905=ORIENTED_EDGE('',*,*,#5137,.T.);
#6906=ORIENTED_EDGE('',*,*,#5154,.T.);
#6907=ORIENTED_EDGE('',*,*,#5110,.T.);
#6908=ORIENTED_EDGE('',*,*,#5136,.T.);
#6909=ORIENTED_EDGE('',*,*,#5114,.T.);
#6910=ORIENTED_EDGE('',*,*,#5152,.T.);
#6911=ORIENTED_EDGE('',*,*,#5170,.F.);
#6912=ORIENTED_EDGE('',*,*,#5131,.F.);
#6913=ORIENTED_EDGE('',*,*,#5171,.F.);
#6914=ORIENTED_EDGE('',*,*,#5169,.F.);
#6915=ORIENTED_EDGE('',*,*,#5171,.T.);
#6916=ORIENTED_EDGE('',*,*,#5151,.F.);
#6917=ORIENTED_EDGE('',*,*,#5172,.F.);
#6918=ORIENTED_EDGE('',*,*,#5166,.F.);
#6919=ORIENTED_EDGE('',*,*,#5170,.T.);
#6920=ORIENTED_EDGE('',*,*,#5168,.F.);
#6921=ORIENTED_EDGE('',*,*,#5173,.F.);
#6922=ORIENTED_EDGE('',*,*,#5150,.F.);
#6923=ORIENTED_EDGE('',*,*,#5172,.T.);
#6924=ORIENTED_EDGE('',*,*,#5145,.F.);
#6925=ORIENTED_EDGE('',*,*,#5173,.T.);
#6926=ORIENTED_EDGE('',*,*,#5167,.F.);
#10029=CYLINDRICAL_SURFACE('',#10966,2.5);
#10030=CYLINDRICAL_SURFACE('',#10969,2.5);
#10031=CYLINDRICAL_SURFACE('',#10972,2.5);
#10032=CYLINDRICAL_SURFACE('',#10975,2.5);
#10033=CYLINDRICAL_SURFACE('',#10978,3.);
#10034=CYLINDRICAL_SURFACE('',#10981,2.99999999999999);
#10035=CYLINDRICAL_SURFACE('',#10984,3.);
#10036=CYLINDRICAL_SURFACE('',#10987,3.);
#10037=CYLINDRICAL_SURFACE('',#10990,3.);
#10038=CYLINDRICAL_SURFACE('',#10993,3.);
#10039=CYLINDRICAL_SURFACE('',#10996,17.5);
#10040=CYLINDRICAL_SURFACE('',#11027,17.5);
#10041=CYLINDRICAL_SURFACE('',#11028,2.50000000000001);
#10042=CYLINDRICAL_SURFACE('',#11029,2.5);
#10043=CYLINDRICAL_SURFACE('',#11030,17.5);
#10044=CYLINDRICAL_SURFACE('',#11031,2.50000000000001);
#10045=CYLINDRICAL_SURFACE('',#11032,2.5);
#10046=CYLINDRICAL_SURFACE('',#11033,3.);
#10047=CYLINDRICAL_SURFACE('',#11036,3.);
#10048=CYLINDRICAL_SURFACE('',#11038,3.);
#10049=CYLINDRICAL_SURFACE('',#11040,3.);
#10210=ADVANCED_FACE('',(#1565),#10029,.F.);
#10211=ADVANCED_FACE('',(#1566),#10030,.F.);
#10212=ADVANCED_FACE('',(#1567),#10031,.F.);
#10213=ADVANCED_FACE('',(#1568),#10032,.F.);
#10214=ADVANCED_FACE('',(#1569),#10033,.F.);
#10215=ADVANCED_FACE('',(#1570),#10034,.F.);
#10216=ADVANCED_FACE('',(#1571),#10035,.F.);
#10217=ADVANCED_FACE('',(#1572),#10036,.F.);
#10218=ADVANCED_FACE('',(#1573),#10037,.F.);
#10219=ADVANCED_FACE('',(#1574),#10038,.F.);
#10220=ADVANCED_FACE('',(#1575),#10039,.F.);
#10221=ADVANCED_FACE('',(#1576),#1465,.T.);
#10222=ADVANCED_FACE('',(#1577),#1466,.T.);
#10223=ADVANCED_FACE('',(#1578),#1467,.T.);
#10224=ADVANCED_FACE('',(#1579),#1468,.T.);
#10225=ADVANCED_FACE('',(#1580),#1469,.T.);
#10226=ADVANCED_FACE('',(#1581,#1377,#1378),#1470,.F.);
#10227=ADVANCED_FACE('',(#1582),#1471,.T.);
#10228=ADVANCED_FACE('',(#1583,#1379,#1380),#1472,.F.);
#10229=ADVANCED_FACE('',(#1584),#1473,.F.);
#10230=ADVANCED_FACE('',(#1585),#1474,.F.);
#10231=ADVANCED_FACE('',(#1586,#1381,#1382),#1475,.T.);
#10232=ADVANCED_FACE('',(#1587),#1476,.T.);
#10233=ADVANCED_FACE('',(#1588,#1383,#1384),#1477,.T.);
#10234=ADVANCED_FACE('',(#1589),#1478,.T.);
#10235=ADVANCED_FACE('',(#1590,#1385,#1386,#1387,#1388,#1389,#1390,#1391),
#1479,.F.);
#10236=ADVANCED_FACE('',(#1591,#1392,#1393,#1394,#1395,#1396,#1397,#1398),
#1480,.T.);
#10237=ADVANCED_FACE('',(#1592),#10040,.F.);
#10238=ADVANCED_FACE('',(#1593),#10041,.F.);
#10239=ADVANCED_FACE('',(#1594),#10042,.F.);
#10240=ADVANCED_FACE('',(#1595),#10043,.F.);
#10241=ADVANCED_FACE('',(#1596),#10044,.F.);
#10242=ADVANCED_FACE('',(#1597),#10045,.F.);
#10243=ADVANCED_FACE('',(#1598),#10046,.T.);
#10244=ADVANCED_FACE('',(#1599),#10047,.T.);
#10245=ADVANCED_FACE('',(#1600),#10048,.T.);
#10246=ADVANCED_FACE('',(#1601),#10049,.T.);
#10819=CLOSED_SHELL('',(#10210,#10211,#10212,#10213,#10214,#10215,#10216,
#10217,#10218,#10219,#10220,#10221,#10222,#10223,#10224,#10225,#10226,#10227,
#10228,#10229,#10230,#10231,#10232,#10233,#10234,#10235,#10236,#10237,#10238,
#10239,#10240,#10241,#10242,#10243,#10244,#10245,#10246));
#10965=AXIS2_PLACEMENT_3D('',#14044,#11892,#11893);
#10966=AXIS2_PLACEMENT_3D('',#14045,#11894,#11895);
#10967=AXIS2_PLACEMENT_3D('',#14047,#11896,#11897);
#10968=AXIS2_PLACEMENT_3D('',#14050,#11899,#11900);
#10969=AXIS2_PLACEMENT_3D('',#14051,#11901,#11902);
#10970=AXIS2_PLACEMENT_3D('',#14053,#11903,#11904);
#10971=AXIS2_PLACEMENT_3D('',#14056,#11906,#11907);
#10972=AXIS2_PLACEMENT_3D('',#14057,#11908,#11909);
#10973=AXIS2_PLACEMENT_3D('',#14059,#11910,#11911);
#10974=AXIS2_PLACEMENT_3D('',#14062,#11913,#11914);
#10975=AXIS2_PLACEMENT_3D('',#14063,#11915,#11916);
#10976=AXIS2_PLACEMENT_3D('',#14065,#11917,#11918);
#10977=AXIS2_PLACEMENT_3D('',#14068,#11920,#11921);
#10978=AXIS2_PLACEMENT_3D('',#14069,#11922,#11923);
#10979=AXIS2_PLACEMENT_3D('',#14071,#11924,#11925);
#10980=AXIS2_PLACEMENT_3D('',#14074,#11927,#11928);
#10981=AXIS2_PLACEMENT_3D('',#14075,#11929,#11930);
#10982=AXIS2_PLACEMENT_3D('',#14077,#11931,#11932);
#10983=AXIS2_PLACEMENT_3D('',#14080,#11934,#11935);
#10984=AXIS2_PLACEMENT_3D('',#14081,#11936,#11937);
#10985=AXIS2_PLACEMENT_3D('',#14083,#11938,#11939);
#10986=AXIS2_PLACEMENT_3D('',#14086,#11941,#11942);
#10987=AXIS2_PLACEMENT_3D('',#14087,#11943,#11944);
#10988=AXIS2_PLACEMENT_3D('',#14089,#11945,#11946);
#10989=AXIS2_PLACEMENT_3D('',#14092,#11948,#11949);
#10990=AXIS2_PLACEMENT_3D('',#14093,#11950,#11951);
#10991=AXIS2_PLACEMENT_3D('',#14095,#11952,#11953);
#10992=AXIS2_PLACEMENT_3D('',#14098,#11955,#11956);
#10993=AXIS2_PLACEMENT_3D('',#14099,#11957,#11958);
#10994=AXIS2_PLACEMENT_3D('',#14101,#11959,#11960);
#10995=AXIS2_PLACEMENT_3D('',#14104,#11962,#11963);
#10996=AXIS2_PLACEMENT_3D('',#14105,#11964,#11965);
#10997=AXIS2_PLACEMENT_3D('',#14107,#11966,#11967);
#10998=AXIS2_PLACEMENT_3D('',#14110,#11969,#11970);
#10999=AXIS2_PLACEMENT_3D('',#14111,#11971,#11972);
#11000=AXIS2_PLACEMENT_3D('',#14128,#11981,#11982);
#11001=AXIS2_PLACEMENT_3D('',#14137,#11987,#11988);
#11002=AXIS2_PLACEMENT_3D('',#14146,#11993,#11994);
#11003=AXIS2_PLACEMENT_3D('',#14155,#11999,#12000);
#11004=AXIS2_PLACEMENT_3D('',#14164,#12005,#12006);
#11005=AXIS2_PLACEMENT_3D('',#14173,#12011,#12012);
#11006=AXIS2_PLACEMENT_3D('',#14174,#12013,#12014);
#11007=AXIS2_PLACEMENT_3D('',#14175,#12015,#12016);
#11008=AXIS2_PLACEMENT_3D('',#14176,#12017,#12018);
#11009=AXIS2_PLACEMENT_3D('',#14190,#12026,#12027);
#11010=AXIS2_PLACEMENT_3D('',#14196,#12031,#12032);
#11011=AXIS2_PLACEMENT_3D('',#14197,#12033,#12034);
#11012=AXIS2_PLACEMENT_3D('',#14198,#12035,#12036);
#11013=AXIS2_PLACEMENT_3D('',#14199,#12037,#12038);
#11014=AXIS2_PLACEMENT_3D('',#14201,#12040,#12041);
#11015=AXIS2_PLACEMENT_3D('',#14203,#12043,#12044);
#11016=AXIS2_PLACEMENT_3D('',#14204,#12045,#12046);
#11017=AXIS2_PLACEMENT_3D('',#14205,#12047,#12048);
#11018=AXIS2_PLACEMENT_3D('',#14206,#12049,#12050);
#11019=AXIS2_PLACEMENT_3D('',#14212,#12054,#12055);
#11020=AXIS2_PLACEMENT_3D('',#14216,#12058,#12059);
#11021=AXIS2_PLACEMENT_3D('',#14217,#12060,#12061);
#11022=AXIS2_PLACEMENT_3D('',#14221,#12064,#12065);
#11023=AXIS2_PLACEMENT_3D('',#14222,#12066,#12067);
#11024=AXIS2_PLACEMENT_3D('',#14223,#12068,#12069);
#11025=AXIS2_PLACEMENT_3D('',#14225,#12071,#12072);
#11026=AXIS2_PLACEMENT_3D('',#14226,#12073,#12074);
#11027=AXIS2_PLACEMENT_3D('',#14235,#12079,#12080);
#11028=AXIS2_PLACEMENT_3D('',#14236,#12081,#12082);
#11029=AXIS2_PLACEMENT_3D('',#14237,#12083,#12084);
#11030=AXIS2_PLACEMENT_3D('',#14238,#12085,#12086);
#11031=AXIS2_PLACEMENT_3D('',#14239,#12087,#12088);
#11032=AXIS2_PLACEMENT_3D('',#14240,#12089,#12090);
#11033=AXIS2_PLACEMENT_3D('',#14241,#12091,#12092);
#11034=AXIS2_PLACEMENT_3D('',#14242,#12093,#12094);
#11035=AXIS2_PLACEMENT_3D('',#14243,#12095,#12096);
#11036=AXIS2_PLACEMENT_3D('',#14244,#12097,#12098);
#11037=AXIS2_PLACEMENT_3D('',#14245,#12099,#12100);
#11038=AXIS2_PLACEMENT_3D('',#14246,#12101,#12102);
#11039=AXIS2_PLACEMENT_3D('',#14247,#12103,#12104);
#11040=AXIS2_PLACEMENT_3D('',#14248,#12105,#12106);
#11892=DIRECTION('axis',(0.,0.,1.));
#11893=DIRECTION('refdir',(1.,0.,0.));
#11894=DIRECTION('center_axis',(1.,0.,0.));
#11895=DIRECTION('ref_axis',(0.,0.,-1.));
#11896=DIRECTION('center_axis',(-1.,0.,0.));
#11897=DIRECTION('ref_axis',(0.,0.,1.));
#11898=DIRECTION('',(1.,0.,0.));
#11899=DIRECTION('center_axis',(1.,0.,0.));
#11900=DIRECTION('ref_axis',(0.,0.,-1.));
#11901=DIRECTION('center_axis',(1.,0.,0.));
#11902=DIRECTION('ref_axis',(0.,0.,-1.));
#11903=DIRECTION('center_axis',(-1.,0.,0.));
#11904=DIRECTION('ref_axis',(0.,0.,1.));
#11905=DIRECTION('',(1.,0.,0.));
#11906=DIRECTION('center_axis',(1.,0.,0.));
#11907=DIRECTION('ref_axis',(0.,0.,-1.));
#11908=DIRECTION('center_axis',(1.,0.,0.));
#11909=DIRECTION('ref_axis',(0.,0.,-1.));
#11910=DIRECTION('center_axis',(1.,0.,0.));
#11911=DIRECTION('ref_axis',(0.,0.,-1.));
#11912=DIRECTION('',(1.,0.,0.));
#11913=DIRECTION('center_axis',(1.,0.,0.));
#11914=DIRECTION('ref_axis',(0.,0.,-1.));
#11915=DIRECTION('center_axis',(1.,0.,0.));
#11916=DIRECTION('ref_axis',(0.,0.,-1.));
#11917=DIRECTION('center_axis',(1.,0.,0.));
#11918=DIRECTION('ref_axis',(0.,0.,-1.));
#11919=DIRECTION('',(1.,0.,0.));
#11920=DIRECTION('center_axis',(1.,0.,0.));
#11921=DIRECTION('ref_axis',(0.,0.,-1.));
#11922=DIRECTION('center_axis',(0.,0.,1.));
#11923=DIRECTION('ref_axis',(1.,0.,0.));
#11924=DIRECTION('center_axis',(0.,0.,1.));
#11925=DIRECTION('ref_axis',(1.,0.,0.));
#11926=DIRECTION('',(0.,0.,1.));
#11927=DIRECTION('center_axis',(0.,0.,1.));
#11928=DIRECTION('ref_axis',(1.,0.,0.));
#11929=DIRECTION('center_axis',(0.,0.,1.));
#11930=DIRECTION('ref_axis',(1.,0.,0.));
#11931=DIRECTION('center_axis',(0.,0.,1.));
#11932=DIRECTION('ref_axis',(1.,0.,0.));
#11933=DIRECTION('',(0.,0.,1.));
#11934=DIRECTION('center_axis',(0.,0.,1.));
#11935=DIRECTION('ref_axis',(1.,0.,0.));
#11936=DIRECTION('center_axis',(0.,0.,1.));
#11937=DIRECTION('ref_axis',(1.,0.,0.));
#11938=DIRECTION('center_axis',(0.,0.,1.));
#11939=DIRECTION('ref_axis',(1.,0.,0.));
#11940=DIRECTION('',(0.,0.,1.));
#11941=DIRECTION('center_axis',(0.,0.,1.));
#11942=DIRECTION('ref_axis',(1.,0.,0.));
#11943=DIRECTION('center_axis',(0.,0.,1.));
#11944=DIRECTION('ref_axis',(1.,0.,0.));
#11945=DIRECTION('center_axis',(0.,0.,1.));
#11946=DIRECTION('ref_axis',(1.,0.,0.));
#11947=DIRECTION('',(0.,0.,1.));
#11948=DIRECTION('center_axis',(0.,0.,1.));
#11949=DIRECTION('ref_axis',(1.,0.,0.));
#11950=DIRECTION('center_axis',(0.,0.,1.));
#11951=DIRECTION('ref_axis',(1.,0.,0.));
#11952=DIRECTION('center_axis',(0.,0.,1.));
#11953=DIRECTION('ref_axis',(1.,0.,0.));
#11954=DIRECTION('',(0.,0.,1.));
#11955=DIRECTION('center_axis',(0.,0.,1.));
#11956=DIRECTION('ref_axis',(1.,0.,0.));
#11957=DIRECTION('center_axis',(0.,0.,1.));
#11958=DIRECTION('ref_axis',(1.,0.,0.));
#11959=DIRECTION('center_axis',(0.,0.,1.));
#11960=DIRECTION('ref_axis',(1.,0.,0.));
#11961=DIRECTION('',(0.,0.,1.));
#11962=DIRECTION('center_axis',(0.,0.,1.));
#11963=DIRECTION('ref_axis',(1.,0.,0.));
#11964=DIRECTION('center_axis',(0.,0.,1.));
#11965=DIRECTION('ref_axis',(1.,0.,0.));
#11966=DIRECTION('center_axis',(0.,0.,1.));
#11967=DIRECTION('ref_axis',(1.,0.,0.));
#11968=DIRECTION('',(0.,0.,1.));
#11969=DIRECTION('center_axis',(0.,0.,1.));
#11970=DIRECTION('ref_axis',(1.,0.,0.));
#11971=DIRECTION('center_axis',(0.,0.,-1.));
#11972=DIRECTION('ref_axis',(-1.,0.,0.));
#11973=DIRECTION('',(1.,0.,0.));
#11974=DIRECTION('',(0.,-1.,0.));
#11975=DIRECTION('',(-1.,0.,0.));
#11976=DIRECTION('',(0.,1.,0.));
#11977=DIRECTION('',(1.,0.,0.));
#11978=DIRECTION('',(0.,1.,0.));
#11979=DIRECTION('',(-1.,0.,0.));
#11980=DIRECTION('',(0.,-1.,0.));
#11981=DIRECTION('center_axis',(0.,0.,-1.));
#11982=DIRECTION('ref_axis',(-1.,0.,0.));
#11983=DIRECTION('',(-1.,0.,0.));
#11984=DIRECTION('',(0.,1.,0.));
#11985=DIRECTION('',(1.,0.,0.));
#11986=DIRECTION('',(0.,1.,0.));
#11987=DIRECTION('center_axis',(0.,0.,-1.));
#11988=DIRECTION('ref_axis',(-1.,0.,0.));
#11989=DIRECTION('',(1.,0.,0.));
#11990=DIRECTION('',(0.,1.,0.));
#11991=DIRECTION('',(-1.,0.,0.));
#11992=DIRECTION('',(0.,1.,0.));
#11993=DIRECTION('center_axis',(0.,0.,-1.));
#11994=DIRECTION('ref_axis',(-1.,0.,0.));
#11995=DIRECTION('',(1.,0.,0.));
#11996=DIRECTION('',(0.,-1.,0.));
#11997=DIRECTION('',(-1.,0.,0.));
#11998=DIRECTION('',(0.,-1.,0.));
#11999=DIRECTION('center_axis',(0.,0.,-1.));
#12000=DIRECTION('ref_axis',(-1.,0.,0.));
#12001=DIRECTION('',(-1.,0.,0.));
#12002=DIRECTION('',(0.,-1.,0.));
#12003=DIRECTION('',(1.,0.,0.));
#12004=DIRECTION('',(0.,-1.,0.));
#12005=DIRECTION('center_axis',(-1.,0.,0.));
#12006=DIRECTION('ref_axis',(0.,0.,1.));
#12007=DIRECTION('',(0.,0.,-1.));
#12008=DIRECTION('',(0.,-1.,0.));
#12009=DIRECTION('',(0.,0.,-1.));
#12010=DIRECTION('',(0.,1.,0.));
#12011=DIRECTION('center_axis',(1.,0.,0.));
#12012=DIRECTION('ref_axis',(0.,0.,-1.));
#12013=DIRECTION('center_axis',(1.,0.,0.));
#12014=DIRECTION('ref_axis',(0.,0.,-1.));
#12015=DIRECTION('center_axis',(1.,0.,0.));
#12016=DIRECTION('ref_axis',(0.,0.,-1.));
#12017=DIRECTION('center_axis',(0.,0.,-1.));
#12018=DIRECTION('ref_axis',(-1.,0.,0.));
#12019=DIRECTION('',(-1.,0.,0.));
#12020=DIRECTION('',(1.,0.,0.));
#12021=DIRECTION('',(0.,-1.,0.));
#12022=DIRECTION('',(-1.,0.,0.));
#12023=DIRECTION('',(0.,-1.,0.));
#12024=DIRECTION('',(1.,-1.33440267382831E-16,0.));
#12025=DIRECTION('',(0.,1.,0.));
#12026=DIRECTION('center_axis',(1.,0.,0.));
#12027=DIRECTION('ref_axis',(0.,0.,-1.));
#12028=DIRECTION('',(0.,0.,-1.));
#12029=DIRECTION('',(0.,1.,0.));
#12030=DIRECTION('',(0.,0.,-1.));
#12031=DIRECTION('center_axis',(1.,0.,0.));
#12032=DIRECTION('ref_axis',(0.,0.,-1.));
#12033=DIRECTION('center_axis',(1.,0.,0.));
#12034=DIRECTION('ref_axis',(0.,0.,-1.));
#12035=DIRECTION('center_axis',(1.,0.,0.));
#12036=DIRECTION('ref_axis',(0.,0.,-1.));
#12037=DIRECTION('center_axis',(0.,1.,0.));
#12038=DIRECTION('ref_axis',(0.,0.,1.));
#12039=DIRECTION('',(-1.,0.,0.));
#12040=DIRECTION('center_axis',(0.,-1.,0.));
#12041=DIRECTION('ref_axis',(0.,0.,-1.));
#12042=DIRECTION('',(1.,0.,0.));
#12043=DIRECTION('center_axis',(-1.,0.,0.));
#12044=DIRECTION('ref_axis',(0.,0.,1.));
#12045=DIRECTION('center_axis',(-1.,0.,0.));
#12046=DIRECTION('ref_axis',(0.,0.,1.));
#12047=DIRECTION('center_axis',(-1.,0.,0.));
#12048=DIRECTION('ref_axis',(0.,0.,1.));
#12049=DIRECTION('center_axis',(-1.,0.,0.));
#12050=DIRECTION('ref_axis',(0.,0.,1.));
#12051=DIRECTION('',(0.,0.,-1.));
#12052=DIRECTION('',(0.,1.,0.));
#12053=DIRECTION('',(0.,0.,-1.));
#12054=DIRECTION('center_axis',(0.,-1.,0.));
#12055=DIRECTION('ref_axis',(0.,0.,-1.));
#12056=DIRECTION('',(-1.,0.,0.));
#12057=DIRECTION('',(0.,0.,-1.));
#12058=DIRECTION('center_axis',(1.,0.,0.));
#12059=DIRECTION('ref_axis',(0.,0.,-1.));
#12060=DIRECTION('center_axis',(1.,0.,0.));
#12061=DIRECTION('ref_axis',(0.,0.,-1.));
#12062=DIRECTION('',(0.,-1.,0.));
#12063=DIRECTION('',(0.,0.,-1.));
#12064=DIRECTION('center_axis',(1.,0.,0.));
#12065=DIRECTION('ref_axis',(0.,0.,-1.));
#12066=DIRECTION('center_axis',(1.,0.,0.));
#12067=DIRECTION('ref_axis',(0.,0.,-1.));
#12068=DIRECTION('center_axis',(1.33440267382831E-16,1.,0.));
#12069=DIRECTION('ref_axis',(-1.,1.33440267382831E-16,0.));
#12070=DIRECTION('',(1.,-1.33440267382831E-16,0.));
#12071=DIRECTION('center_axis',(0.,0.,1.));
#12072=DIRECTION('ref_axis',(1.,0.,0.));
#12073=DIRECTION('center_axis',(0.,0.,1.));
#12074=DIRECTION('ref_axis',(1.,0.,0.));
#12075=DIRECTION('',(-1.,0.,0.));
#12076=DIRECTION('',(0.,-1.,0.));
#12077=DIRECTION('',(1.,0.,0.));
#12078=DIRECTION('',(0.,1.,0.));
#12079=DIRECTION('center_axis',(1.,0.,0.));
#12080=DIRECTION('ref_axis',(0.,1.22464679914735E-16,1.));
#12081=DIRECTION('center_axis',(1.,0.,0.));
#12082=DIRECTION('ref_axis',(0.,1.22464679914735E-16,1.));
#12083=DIRECTION('center_axis',(1.,0.,0.));
#12084=DIRECTION('ref_axis',(0.,1.22464679914735E-16,1.));
#12085=DIRECTION('center_axis',(1.,0.,0.));
#12086=DIRECTION('ref_axis',(0.,1.22464679914735E-16,1.));
#12087=DIRECTION('center_axis',(1.,0.,0.));
#12088=DIRECTION('ref_axis',(0.,1.22464679914735E-16,1.));
#12089=DIRECTION('center_axis',(1.,0.,0.));
#12090=DIRECTION('ref_axis',(0.,1.22464679914735E-16,1.));
#12091=DIRECTION('center_axis',(0.,-1.,0.));
#12092=DIRECTION('ref_axis',(0.,0.,-1.));
#12093=DIRECTION('center_axis',(-0.707106781186549,-0.707106781186546,-1.50457204420145E-15));
#12094=DIRECTION('ref_axis',(0.707106781186546,-0.707106781186549,-9.86517477994685E-14));
#12095=DIRECTION('center_axis',(-0.707106781186548,0.707106781186548,0.));
#12096=DIRECTION('ref_axis',(0.707106781186548,0.707106781186548,-2.92621452477431E-13));
#12097=DIRECTION('center_axis',(1.,0.,0.));
#12098=DIRECTION('ref_axis',(0.,0.,-1.));
#12099=DIRECTION('center_axis',(-0.70710678118655,-0.707106781186545,5.06083323958671E-15));
#12100=DIRECTION('ref_axis',(0.707106781186545,-0.70710678118655,1.41538849381609E-13));
#12101=DIRECTION('center_axis',(-1.,0.,0.));
#12102=DIRECTION('ref_axis',(0.,0.,1.));
#12103=DIRECTION('center_axis',(-0.707106781186552,0.707106781186543,6.56540528378815E-15));
#12104=DIRECTION('ref_axis',(0.707106781186543,0.707106781186552,2.52973120306771E-13));
#12105=DIRECTION('center_axis',(0.,1.,0.));
#12106=DIRECTION('ref_axis',(0.,0.,1.));
#14044=CARTESIAN_POINT('',(0.,0.,0.));
#14045=CARTESIAN_POINT('Origin',(-62.,46.68,3.68653347947321));
#14046=CARTESIAN_POINT('',(52.,46.68,6.18653347947322));
#14047=CARTESIAN_POINT('Origin',(52.,46.68,3.68653347947321));
#14048=CARTESIAN_POINT('',(62.,46.68,6.18653347947322));
#14049=CARTESIAN_POINT('',(-62.,46.68,6.18653347947322));
#14050=CARTESIAN_POINT('Origin',(62.,46.68,3.68653347947321));
#14051=CARTESIAN_POINT('Origin',(-62.,25.68,3.68653347947321));
#14052=CARTESIAN_POINT('',(52.,25.68,6.18653347947322));
#14053=CARTESIAN_POINT('Origin',(52.,25.68,3.68653347947321));
#14054=CARTESIAN_POINT('',(62.,25.68,6.18653347947322));
#14055=CARTESIAN_POINT('',(-62.,25.68,6.18653347947322));
#14056=CARTESIAN_POINT('Origin',(62.,25.68,3.68653347947321));
#14057=CARTESIAN_POINT('Origin',(-62.,46.68,3.68653347947321));
#14058=CARTESIAN_POINT('',(-62.,46.68,6.18653347947322));
#14059=CARTESIAN_POINT('Origin',(-62.,46.68,3.68653347947321));
#14060=CARTESIAN_POINT('',(-52.,46.68,6.18653347947322));
#14061=CARTESIAN_POINT('',(-62.,46.68,6.18653347947322));
#14062=CARTESIAN_POINT('Origin',(-52.,46.68,3.68653347947321));
#14063=CARTESIAN_POINT('Origin',(-62.,25.68,3.68653347947321));
#14064=CARTESIAN_POINT('',(-62.,25.68,6.18653347947322));
#14065=CARTESIAN_POINT('Origin',(-62.,25.68,3.68653347947321));
#14066=CARTESIAN_POINT('',(-52.,25.68,6.18653347947322));
#14067=CARTESIAN_POINT('',(-62.,25.68,6.18653347947322));
#14068=CARTESIAN_POINT('Origin',(-52.,25.68,3.68653347947321));
#14069=CARTESIAN_POINT('Origin',(-26.310635094611,-8.00000000000001,14.5));
#14070=CARTESIAN_POINT('',(-29.310635094611,-8.00000000000001,14.5));
#14071=CARTESIAN_POINT('Origin',(-26.310635094611,-8.00000000000001,14.5));
#14072=CARTESIAN_POINT('',(-29.310635094611,-8.00000000000001,24.5));
#14073=CARTESIAN_POINT('',(-29.310635094611,-8.00000000000001,14.5));
#14074=CARTESIAN_POINT('Origin',(-26.310635094611,-8.00000000000001,24.5));
#14075=CARTESIAN_POINT('Origin',(-26.310635094611,-33.,14.5));
#14076=CARTESIAN_POINT('',(-29.310635094611,-33.,14.5));
#14077=CARTESIAN_POINT('Origin',(-26.310635094611,-33.,14.5));
#14078=CARTESIAN_POINT('',(-29.310635094611,-33.,24.5));
#14079=CARTESIAN_POINT('',(-29.310635094611,-33.,14.5));
#14080=CARTESIAN_POINT('Origin',(-26.310635094611,-33.,24.5));
#14081=CARTESIAN_POINT('Origin',(-4.66,-45.5,14.5));
#14082=CARTESIAN_POINT('',(-7.66000000000001,-45.5,14.5));
#14083=CARTESIAN_POINT('Origin',(-4.66,-45.5,14.5));
#14084=CARTESIAN_POINT('',(-7.66000000000001,-45.5,24.5));
#14085=CARTESIAN_POINT('',(-7.66000000000001,-45.5,14.5));
#14086=CARTESIAN_POINT('Origin',(-4.66,-45.5,24.5));
#14087=CARTESIAN_POINT('Origin',(16.990635094611,-33.,14.5));
#14088=CARTESIAN_POINT('',(13.990635094611,-33.,14.5));
#14089=CARTESIAN_POINT('Origin',(16.990635094611,-33.,14.5));
#14090=CARTESIAN_POINT('',(13.990635094611,-33.,24.5));
#14091=CARTESIAN_POINT('',(13.990635094611,-33.,14.5));
#14092=CARTESIAN_POINT('Origin',(16.990635094611,-33.,24.5));
#14093=CARTESIAN_POINT('Origin',(16.990635094611,-8.00000000000001,14.5));
#14094=CARTESIAN_POINT('',(13.990635094611,-8.00000000000001,14.5));
#14095=CARTESIAN_POINT('Origin',(16.990635094611,-8.00000000000001,14.5));
#14096=CARTESIAN_POINT('',(13.990635094611,-8.00000000000001,24.5));
#14097=CARTESIAN_POINT('',(13.990635094611,-8.00000000000001,14.5));
#14098=CARTESIAN_POINT('Origin',(16.990635094611,-8.00000000000001,24.5));
#14099=CARTESIAN_POINT('Origin',(-4.66,4.49999999999999,14.5));
#14100=CARTESIAN_POINT('',(-7.66,4.49999999999999,14.5));
#14101=CARTESIAN_POINT('Origin',(-4.66,4.49999999999999,14.5));
#14102=CARTESIAN_POINT('',(-7.66,4.49999999999999,24.5));
#14103=CARTESIAN_POINT('',(-7.66,4.49999999999999,14.5));
#14104=CARTESIAN_POINT('Origin',(-4.66,4.49999999999999,24.5));
#14105=CARTESIAN_POINT('Origin',(-4.66,-20.5,14.5));
#14106=CARTESIAN_POINT('',(-22.16,-20.5,14.5));
#14107=CARTESIAN_POINT('Origin',(-4.66,-20.5,14.5));
#14108=CARTESIAN_POINT('',(-22.16,-20.5,24.5));
#14109=CARTESIAN_POINT('',(-22.16,-20.5,14.5));
#14110=CARTESIAN_POINT('Origin',(-4.66,-20.5,24.5));
#14111=CARTESIAN_POINT('Origin',(0.,0.,-14.5));
#14112=CARTESIAN_POINT('',(-62.,59.68,-14.5));
#14113=CARTESIAN_POINT('',(-52.,59.68,-14.5));
#14114=CARTESIAN_POINT('',(-62.,59.68,-14.5));
#14115=CARTESIAN_POINT('',(-62.,76.5,-14.5));
#14116=CARTESIAN_POINT('',(-62.,-76.5,-14.5));
#14117=CARTESIAN_POINT('',(62.,76.5,-14.5));
#14118=CARTESIAN_POINT('',(-62.,76.5,-14.5));
#14119=CARTESIAN_POINT('',(62.,59.68,-14.5));
#14120=CARTESIAN_POINT('',(62.,-76.5,-14.5));
#14121=CARTESIAN_POINT('',(52.,59.68,-14.5));
#14122=CARTESIAN_POINT('',(-62.,59.68,-14.5));
#14123=CARTESIAN_POINT('',(52.,66.5,-14.5));
#14124=CARTESIAN_POINT('',(52.,-66.5,-14.5));
#14125=CARTESIAN_POINT('',(-52.,66.5,-14.5));
#14126=CARTESIAN_POINT('',(-52.,66.5,-14.5));
#14127=CARTESIAN_POINT('',(-52.,-66.5,-14.5));
#14128=CARTESIAN_POINT('Origin',(0.,0.,-14.5));
#14129=CARTESIAN_POINT('',(62.,54.68,-14.5));
#14130=CARTESIAN_POINT('',(52.,54.68,-14.5));
#14131=CARTESIAN_POINT('',(-62.,54.68,-14.5));
#14132=CARTESIAN_POINT('',(62.,53.68,-14.5));
#14133=CARTESIAN_POINT('',(62.,-76.5,-14.5));
#14134=CARTESIAN_POINT('',(52.,53.68,-14.5));
#14135=CARTESIAN_POINT('',(-62.,53.68,-14.5));
#14136=CARTESIAN_POINT('',(52.,-66.5,-14.5));
#14137=CARTESIAN_POINT('Origin',(0.,0.,-14.5));
#14138=CARTESIAN_POINT('',(52.,17.68,-14.5));
#14139=CARTESIAN_POINT('',(62.,17.68,-14.5));
#14140=CARTESIAN_POINT('',(-62.,17.68,-14.5));
#14141=CARTESIAN_POINT('',(52.,18.68,-14.5));
#14142=CARTESIAN_POINT('',(52.,-66.5,-14.5));
#14143=CARTESIAN_POINT('',(62.,18.68,-14.5));
#14144=CARTESIAN_POINT('',(-62.,18.68,-14.5));
#14145=CARTESIAN_POINT('',(62.,-76.5,-14.5));
#14146=CARTESIAN_POINT('Origin',(0.,0.,-14.5));
#14147=CARTESIAN_POINT('',(-62.,17.68,-14.5));
#14148=CARTESIAN_POINT('',(-52.,17.68,-14.5));
#14149=CARTESIAN_POINT('',(-62.,17.68,-14.5));
#14150=CARTESIAN_POINT('',(-62.,18.68,-14.5));
#14151=CARTESIAN_POINT('',(-62.,-76.5,-14.5));
#14152=CARTESIAN_POINT('',(-52.,18.68,-14.5));
#14153=CARTESIAN_POINT('',(-62.,18.68,-14.5));
#14154=CARTESIAN_POINT('',(-52.,-66.5,-14.5));
#14155=CARTESIAN_POINT('Origin',(0.,0.,-14.5));
#14156=CARTESIAN_POINT('',(-52.,54.68,-14.5));
#14157=CARTESIAN_POINT('',(-62.,54.68,-14.5));
#14158=CARTESIAN_POINT('',(-62.,54.68,-14.5));
#14159=CARTESIAN_POINT('',(-52.,53.68,-14.5));
#14160=CARTESIAN_POINT('',(-52.,-66.5,-14.5));
#14161=CARTESIAN_POINT('',(-62.,53.68,-14.5));
#14162=CARTESIAN_POINT('',(-62.,53.68,-14.5));
#14163=CARTESIAN_POINT('',(-62.,-76.5,-14.5));
#14164=CARTESIAN_POINT('Origin',(62.,-76.5,14.5));
#14165=CARTESIAN_POINT('',(62.,76.5,21.5));
#14166=CARTESIAN_POINT('',(62.,76.5,14.5));
#14167=CARTESIAN_POINT('',(62.,-76.5,21.5));
#14168=CARTESIAN_POINT('',(62.,-76.5,21.5));
#14169=CARTESIAN_POINT('',(62.,-76.5,-14.5));
#14170=CARTESIAN_POINT('',(62.,-76.5,14.5));
#14171=CARTESIAN_POINT('',(62.,12.68,-14.5));
#14172=CARTESIAN_POINT('',(62.,-76.5,-14.5));
#14173=CARTESIAN_POINT('Origin',(62.,15.18,-14.5));
#14174=CARTESIAN_POINT('Origin',(62.,36.18,-14.5));
#14175=CARTESIAN_POINT('Origin',(62.,57.18,-14.5));
#14176=CARTESIAN_POINT('Origin',(0.,0.,-14.5));
#14177=CARTESIAN_POINT('',(52.,12.68,-14.5));
#14178=CARTESIAN_POINT('',(-62.,12.68,-14.5));
#14179=CARTESIAN_POINT('',(-62.,-76.5,-14.5));
#14180=CARTESIAN_POINT('',(-62.,-76.5,-14.5));
#14181=CARTESIAN_POINT('',(-62.,12.68,-14.5));
#14182=CARTESIAN_POINT('',(-62.,-76.5,-14.5));
#14183=CARTESIAN_POINT('',(-52.,12.68,-14.5));
#14184=CARTESIAN_POINT('',(-62.,12.68,-14.5));
#14185=CARTESIAN_POINT('',(-52.,-66.5,-14.5));
#14186=CARTESIAN_POINT('',(-52.,-66.5,-14.5));
#14187=CARTESIAN_POINT('',(52.,-66.5,-14.5));
#14188=CARTESIAN_POINT('',(-52.,-66.5,-14.5));
#14189=CARTESIAN_POINT('',(52.,-66.5,-14.5));
#14190=CARTESIAN_POINT('Origin',(-62.,-76.5,14.5));
#14191=CARTESIAN_POINT('',(-62.,-76.5,21.5));
#14192=CARTESIAN_POINT('',(-62.,-76.5,14.5));
#14193=CARTESIAN_POINT('',(-62.,76.5,21.5));
#14194=CARTESIAN_POINT('',(-62.,76.5,21.5));
#14195=CARTESIAN_POINT('',(-62.,76.5,14.5));
#14196=CARTESIAN_POINT('Origin',(-62.,57.18,-14.5));
#14197=CARTESIAN_POINT('Origin',(-62.,36.18,-14.5));
#14198=CARTESIAN_POINT('Origin',(-62.,15.18,-14.5));
#14199=CARTESIAN_POINT('Origin',(-62.,-76.5,14.5));
#14200=CARTESIAN_POINT('',(-62.,-76.5,21.5));
#14201=CARTESIAN_POINT('Origin',(-62.,76.5,14.5));
#14202=CARTESIAN_POINT('',(62.,76.5,21.5));
#14203=CARTESIAN_POINT('Origin',(52.,-66.5,14.5));
#14204=CARTESIAN_POINT('Origin',(52.,57.18,-14.5));
#14205=CARTESIAN_POINT('Origin',(52.,36.18,-14.5));
#14206=CARTESIAN_POINT('Origin',(52.,15.18,-14.5));
#14207=CARTESIAN_POINT('',(52.,-66.5,14.5));
#14208=CARTESIAN_POINT('',(52.,-66.5,14.5));
#14209=CARTESIAN_POINT('',(52.,66.5,14.5));
#14210=CARTESIAN_POINT('',(52.,-66.5,14.5));
#14211=CARTESIAN_POINT('',(52.,66.5,14.5));
#14212=CARTESIAN_POINT('Origin',(-52.,66.5,14.5));
#14213=CARTESIAN_POINT('',(-52.,66.5,14.5));
#14214=CARTESIAN_POINT('',(-52.,66.5,14.5));
#14215=CARTESIAN_POINT('',(-52.,66.5,14.5));
#14216=CARTESIAN_POINT('Origin',(-52.,-66.5,14.5));
#14217=CARTESIAN_POINT('Origin',(-52.,57.18,-14.5));
#14218=CARTESIAN_POINT('',(-52.,-66.5,14.5));
#14219=CARTESIAN_POINT('',(-52.,-66.5,14.5));
#14220=CARTESIAN_POINT('',(-52.,-66.5,14.5));
#14221=CARTESIAN_POINT('Origin',(-52.,15.18,-14.5));
#14222=CARTESIAN_POINT('Origin',(-52.,36.18,-14.5));
#14223=CARTESIAN_POINT('Origin',(-52.,-66.5,14.5));
#14224=CARTESIAN_POINT('',(-52.,-66.5,14.5));
#14225=CARTESIAN_POINT('Origin',(0.,0.,14.5));
#14226=CARTESIAN_POINT('Origin',(0.,0.,24.5));
#14227=CARTESIAN_POINT('',(59.,73.5,24.5));
#14228=CARTESIAN_POINT('',(-59.,73.5,24.5));
#14229=CARTESIAN_POINT('',(-62.,73.5,24.5));
#14230=CARTESIAN_POINT('',(-59.,-73.5,24.5));
#14231=CARTESIAN_POINT('',(-59.,-76.5,24.5));
#14232=CARTESIAN_POINT('',(59.,-73.5,24.5));
#14233=CARTESIAN_POINT('',(62.,-73.5,24.5));
#14234=CARTESIAN_POINT('',(59.,76.5,24.5));
#14235=CARTESIAN_POINT('Origin',(-62.,36.18,-14.5));
#14236=CARTESIAN_POINT('Origin',(-62.,15.18,-14.5));
#14237=CARTESIAN_POINT('Origin',(-62.,57.18,-14.5));
#14238=CARTESIAN_POINT('Origin',(-62.,36.18,-14.5));
#14239=CARTESIAN_POINT('Origin',(-62.,15.18,-14.5));
#14240=CARTESIAN_POINT('Origin',(-62.,57.18,-14.5));
#14241=CARTESIAN_POINT('Origin',(59.,0.,21.5));
#14242=CARTESIAN_POINT('Origin',(59.0000000000002,-73.5000000000002,21.5000000000003));
#14243=CARTESIAN_POINT('Origin',(59.0000000000008,73.5000000000007,21.5000000000007));
#14244=CARTESIAN_POINT('Origin',(0.,73.5,21.5));
#14245=CARTESIAN_POINT('Origin',(-59.0000000000003,73.5000000000003,21.5000000000004));
#14246=CARTESIAN_POINT('Origin',(0.,-73.5,21.5));
#14247=CARTESIAN_POINT('Origin',(-59.0000000000006,-73.5000000000006,21.5000000000007));
#14248=CARTESIAN_POINT('Origin',(-59.,0.,21.5));
#37855=UNCERTAINTY_MEASURE_WITH_UNIT(LENGTH_MEASURE(0.01),#37882,
'DISTANCE_ACCURACY_VALUE',
'Maximum model space distance between geometric entities at asserted c
onnectivities');
#37867=UNCERTAINTY_MEASURE_WITH_UNIT(LENGTH_MEASURE(0.01),#37882,
'DISTANCE_ACCURACY_VALUE',
'Maximum model space distance between geometric entities at asserted c
onnectivities');
#37869=(
GEOMETRIC_REPRESENTATION_CONTEXT(3)
GLOBAL_UNCERTAINTY_ASSIGNED_CONTEXT((#37855))
GLOBAL_UNIT_ASSIGNED_CONTEXT((#37882,#37884,#37885))
REPRESENTATION_CONTEXT('','3D')
);
#37881=(
GEOMETRIC_REPRESENTATION_CONTEXT(3)
GLOBAL_UNCERTAINTY_ASSIGNED_CONTEXT((#37867))
GLOBAL_UNIT_ASSIGNED_CONTEXT((#37882,#37884,#37885))
REPRESENTATION_CONTEXT('','3D')
);
#37882=(
LENGTH_UNIT()
NAMED_UNIT(*)
SI_UNIT(.MILLI.,.METRE.)
);
#37884=(
NAMED_UNIT(*)
PLANE_ANGLE_UNIT()
SI_UNIT($,.RADIAN.)
);
#37885=(
NAMED_UNIT(*)
SI_UNIT($,.STERADIAN.)
SOLID_ANGLE_UNIT()
);
#37887=SHAPE_DEFINITION_REPRESENTATION(#37900,#37954);
#37900=PRODUCT_DEFINITION_SHAPE('',$,#37968);
#37954=SHAPE_REPRESENTATION('',(#10965),#37869);
#37966=PRODUCT_DEFINITION_CONTEXT('part definition',#38007,'design');
#37968=PRODUCT_DEFINITION('PS01','Body_A',#37981,#37966);
#37981=PRODUCT_DEFINITION_FORMATION('',$,#38010);
#38007=APPLICATION_CONTEXT(
'Core Data for Automotive Mechanical Design Process');
#38008=PRODUCT_CONTEXT('part definition',#38007,'mechanical');
#38010=PRODUCT('PS01','Body_A',$,(#38008));
#38023=PRESENTATION_STYLE_ASSIGNMENT((#38025));
#38025=SURFACE_STYLE_USAGE(.BOTH.,#38027);
#38027=SURFACE_SIDE_STYLE('',(#38029));
#38029=SURFACE_STYLE_FILL_AREA(#38031);
#38031=FILL_AREA_STYLE('Opaque(202,209,238)',(#38033));
#38033=FILL_AREA_STYLE_COLOUR('Opaque(202,209,238)',#38035);
#38035=COLOUR_RGB('Opaque(202,209,238)', 0.66274510, 0.83137255, 0.94901961);
ENDSEC;
END-ISO-10303-21;
